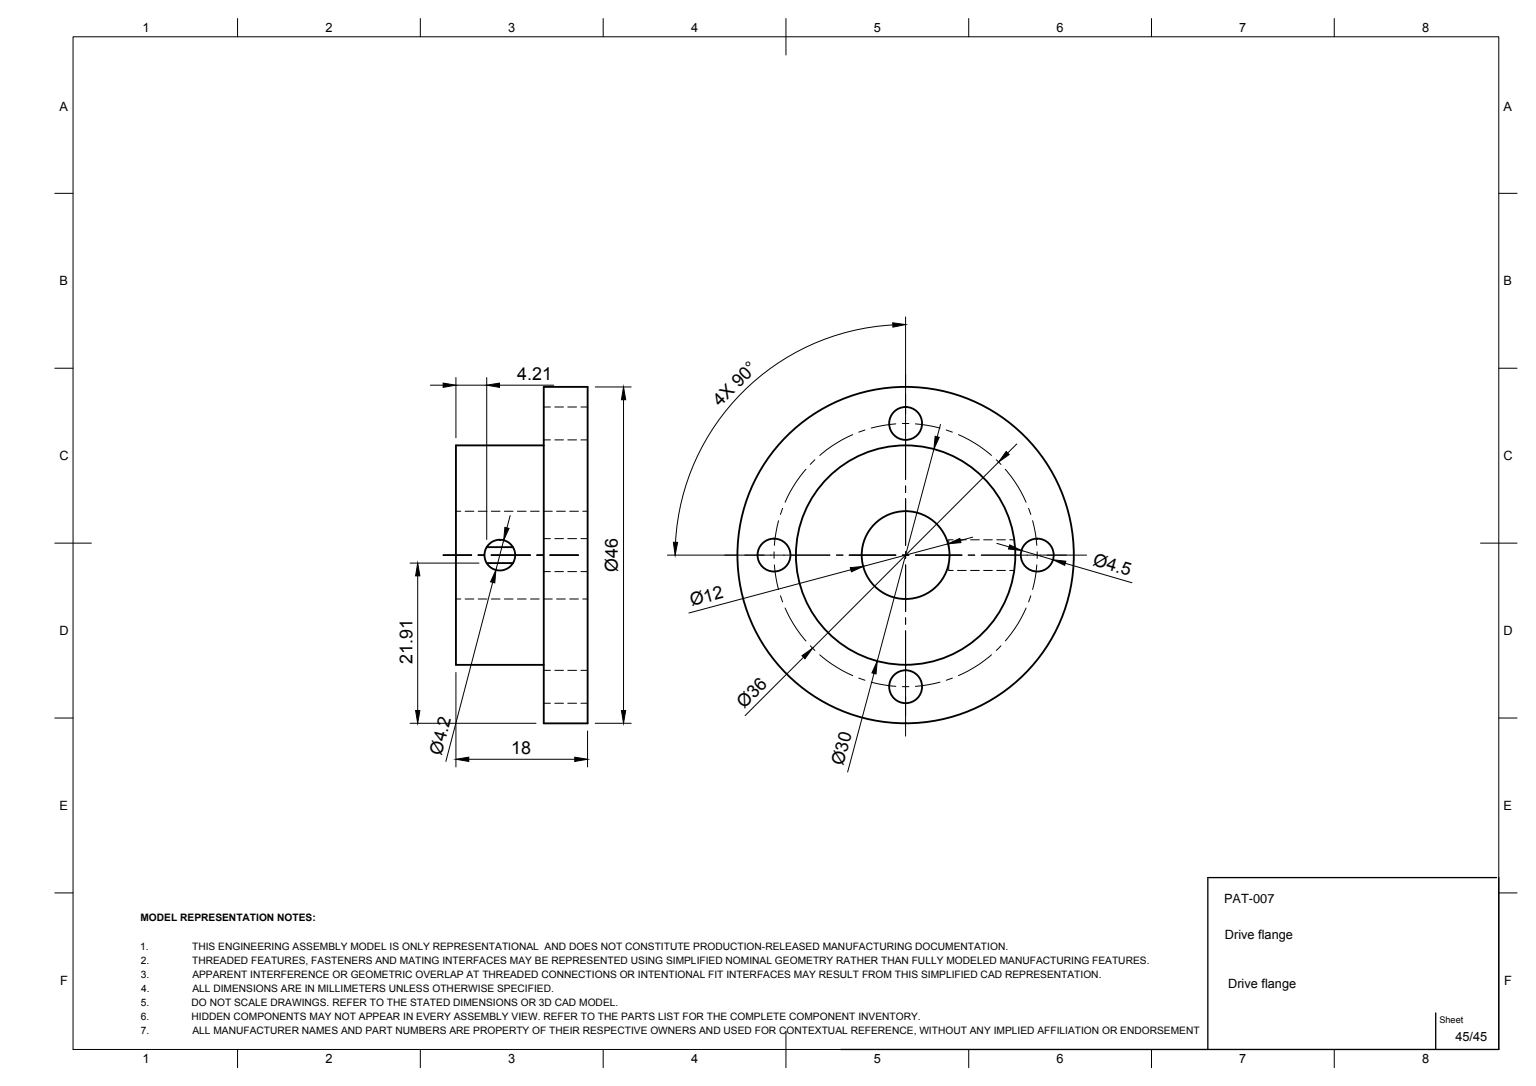
ISO-10303-21;
HEADER;
/* Generated by software containing ST-Developer
 * from STEP Tools, Inc. (www.steptools.com) 
 */

FILE_DESCRIPTION(
/* description */ ('Bearing friction torque test rig'),
/* implementation_level */ '2;1');

FILE_NAME(
/* name */ 'Drive flange.step',
/* time_stamp */ '2026-10-28T03:24:04-07:00',
/* author */ (''),
/* organization */ (''),
/* preprocessor_version */ 'ST-DEVELOPER v20.2',
/* originating_system */ 'Autodesk Translation Framework v15.17.0.0',
/* authorisation */ '');

FILE_SCHEMA (('AUTOMOTIVE_DESIGN { 1 0 10303 214 3 1 1 }'));
ENDSEC;

DATA;
#10=MECHANICAL_DESIGN_GEOMETRIC_PRESENTATION_REPRESENTATION('',(#591),#14822);
#391=B_SPLINE_CURVE_WITH_KNOTS('',3,(#14552,#14553,#14554,#14555,#14556,
#14557,#14558,#14559,#14560,#14561),.UNSPECIFIED.,.F.,.F.,(4,2,2,2,4),(0.847831445683407,
0.87827457693095,0.958092875386316,1.03791117384168,1.06835430508922),
 .UNSPECIFIED.);
#392=B_SPLINE_CURVE_WITH_KNOTS('',3,(#14567,#14568,#14569,#14570,#14571,
#14572,#14573,#14574,#14575,#14576,#14577,#14578,#14579,#14580,#14581,#14582,
#14583,#14584),.UNSPECIFIED.,.F.,.F.,(4,2,2,2,2,2,2,2,4),(0.,0.0792165807733633,
0.158433161546727,0.237648697074571,0.316864232602415,0.396079768130259,
0.475295303658104,0.554511884431467,0.63372846520483),.UNSPECIFIED.);
#393=B_SPLINE_CURVE_WITH_KNOTS('',3,(#14585,#14586,#14587,#14588,#14589,
#14590,#14591,#14592,#14593,#14594,#14595,#14596,#14597,#14598,#14599,#14600,
#14601,#14602),.UNSPECIFIED.,.F.,.F.,(4,2,2,2,2,2,2,2,4),(0.63372846520483,
0.712945045978194,0.792161626751557,0.871377162279401,0.950592697807245,
1.02980823333509,1.10902376886293,1.1882403496363,1.26745693040966),
 .UNSPECIFIED.);
#394=B_SPLINE_CURVE_WITH_KNOTS('',3,(#14605,#14606,#14607,#14608,#14609,
#14610,#14611,#14612,#14613,#14614),.UNSPECIFIED.,.F.,.F.,(4,2,2,2,4),(0.20910286209253,
0.239545993340073,0.319364291795439,0.399182590250804,0.429625721498348),
 .UNSPECIFIED.);
#498=SHAPE_REPRESENTATION_RELATIONSHIP('SRR','None',#15040,#537);
#537=ADVANCED_BREP_SHAPE_REPRESENTATION('',(#642),#14820);
#591=STYLED_ITEM('',(#15277),#642);
#642=MANIFOLD_SOLID_BREP('Body1',#7710);
#860=FACE_BOUND('',#2188,.T.);
#861=FACE_BOUND('',#2189,.T.);
#862=FACE_BOUND('',#2190,.T.);
#863=FACE_BOUND('',#2191,.T.);
#864=FACE_BOUND('',#2192,.T.);
#865=FACE_BOUND('',#2195,.T.);
#866=FACE_BOUND('',#2197,.T.);
#867=FACE_BOUND('',#2199,.T.);
#868=FACE_BOUND('',#2201,.T.);
#869=FACE_BOUND('',#2202,.T.);
#870=FACE_BOUND('',#2203,.T.);
#871=FACE_BOUND('',#2204,.T.);
#872=FACE_BOUND('',#2205,.T.);
#1085=PLANE('',#9102);
#1086=PLANE('',#9107);
#1087=PLANE('',#9120);
#1088=PLANE('',#9130);
#1089=PLANE('',#9131);
#1519=FACE_OUTER_BOUND('',#2180,.T.);
#1520=FACE_OUTER_BOUND('',#2181,.T.);
#1521=FACE_OUTER_BOUND('',#2182,.T.);
#1522=FACE_OUTER_BOUND('',#2183,.T.);
#1523=FACE_OUTER_BOUND('',#2184,.T.);
#1524=FACE_OUTER_BOUND('',#2185,.T.);
#1525=FACE_OUTER_BOUND('',#2186,.T.);
#1526=FACE_OUTER_BOUND('',#2187,.T.);
#1527=FACE_OUTER_BOUND('',#2193,.T.);
#1528=FACE_OUTER_BOUND('',#2194,.T.);
#1529=FACE_OUTER_BOUND('',#2196,.T.);
#1530=FACE_OUTER_BOUND('',#2198,.T.);
#1531=FACE_OUTER_BOUND('',#2200,.T.);
#2180=EDGE_LOOP('',(#6932,#6933));
#2181=EDGE_LOOP('',(#6934,#6935,#6936,#6937,#6938,#6939,#6940,#6941,#6942));
#2182=EDGE_LOOP('',(#6943,#6944,#6945));
#2183=EDGE_LOOP('',(#6946,#6947,#6948,#6949));
#2184=EDGE_LOOP('',(#6950,#6951,#6952,#6953));
#2185=EDGE_LOOP('',(#6954,#6955,#6956,#6957));
#2186=EDGE_LOOP('',(#6958,#6959,#6960,#6961));
#2187=EDGE_LOOP('',(#6962));
#2188=EDGE_LOOP('',(#6963));
#2189=EDGE_LOOP('',(#6964));
#2190=EDGE_LOOP('',(#6965));
#2191=EDGE_LOOP('',(#6966));
#2192=EDGE_LOOP('',(#6967));
#2193=EDGE_LOOP('',(#6968,#6969,#6970,#6971));
#2194=EDGE_LOOP('',(#6972,#6973,#6974,#6975));
#2195=EDGE_LOOP('',(#6976,#6977,#6978,#6979));
#2196=EDGE_LOOP('',(#6980,#6981,#6982,#6983));
#2197=EDGE_LOOP('',(#6984,#6985));
#2198=EDGE_LOOP('',(#6986));
#2199=EDGE_LOOP('',(#6987));
#2200=EDGE_LOOP('',(#6988));
#2201=EDGE_LOOP('',(#6989));
#2202=EDGE_LOOP('',(#6990));
#2203=EDGE_LOOP('',(#6991));
#2204=EDGE_LOOP('',(#6992));
#2205=EDGE_LOOP('',(#6993));
#2632=LINE('',#14548,#3076);
#2633=LINE('',#14565,#3077);
#2634=LINE('',#14616,#3078);
#2635=LINE('',#14621,#3079);
#2636=LINE('',#14627,#3080);
#2637=LINE('',#14633,#3081);
#2638=LINE('',#14639,#3082);
#2639=LINE('',#14648,#3083);
#2640=LINE('',#14654,#3084);
#2641=LINE('',#14659,#3085);
#3076=VECTOR('',#11501,1.);
#3077=VECTOR('',#11508,0.21);
#3078=VECTOR('',#11513,1.);
#3079=VECTOR('',#11518,0.225);
#3080=VECTOR('',#11525,0.225);
#3081=VECTOR('',#11532,0.225);
#3082=VECTOR('',#11539,0.225);
#3083=VECTOR('',#11550,2.3);
#3084=VECTOR('',#11557,0.6);
#3085=VECTOR('',#11564,1.5);
#3532=CIRCLE('',#9103,0.21);
#3533=CIRCLE('',#9105,0.21);
#3534=CIRCLE('',#9106,0.21);
#3535=CIRCLE('',#9109,0.225);
#3536=CIRCLE('',#9110,0.225);
#3537=CIRCLE('',#9112,0.225);
#3538=CIRCLE('',#9113,0.225);
#3539=CIRCLE('',#9115,0.225);
#3540=CIRCLE('',#9116,0.225);
#3541=CIRCLE('',#9118,0.225);
#3542=CIRCLE('',#9119,0.225);
#3543=CIRCLE('',#9121,2.3);
#3544=CIRCLE('',#9122,1.5);
#3545=CIRCLE('',#9124,2.3);
#3546=CIRCLE('',#9126,0.6);
#3547=CIRCLE('',#9127,0.6);
#3548=CIRCLE('',#9129,1.5);
#4163=VERTEX_POINT('',#14546);
#4164=VERTEX_POINT('',#14547);
#4165=VERTEX_POINT('',#14551);
#4166=VERTEX_POINT('',#14562);
#4167=VERTEX_POINT('',#14564);
#4168=VERTEX_POINT('',#14566);
#4169=VERTEX_POINT('',#14603);
#4170=VERTEX_POINT('',#14618);
#4171=VERTEX_POINT('',#14620);
#4172=VERTEX_POINT('',#14624);
#4173=VERTEX_POINT('',#14626);
#4174=VERTEX_POINT('',#14630);
#4175=VERTEX_POINT('',#14632);
#4176=VERTEX_POINT('',#14636);
#4177=VERTEX_POINT('',#14638);
#4178=VERTEX_POINT('',#14642);
#4179=VERTEX_POINT('',#14644);
#4180=VERTEX_POINT('',#14647);
#4181=VERTEX_POINT('',#14651);
#4182=VERTEX_POINT('',#14653);
#4183=VERTEX_POINT('',#14657);
#5092=EDGE_CURVE('',#4163,#4164,#2632,.T.);
#5093=EDGE_CURVE('',#4163,#4164,#3532,.T.);
#5094=EDGE_CURVE('',#4165,#4163,#391,.T.);
#5095=EDGE_CURVE('',#4166,#4165,#3533,.T.);
#5096=EDGE_CURVE('',#4166,#4167,#2633,.T.);
#5097=EDGE_CURVE('',#4168,#4167,#392,.T.);
#5098=EDGE_CURVE('',#4167,#4168,#393,.T.);
#5099=EDGE_CURVE('',#4169,#4166,#3534,.T.);
#5100=EDGE_CURVE('',#4164,#4169,#394,.T.);
#5101=EDGE_CURVE('',#4169,#4165,#2634,.T.);
#5102=EDGE_CURVE('',#4170,#4170,#3535,.T.);
#5103=EDGE_CURVE('',#4170,#4171,#2635,.T.);
#5104=EDGE_CURVE('',#4171,#4171,#3536,.T.);
#5105=EDGE_CURVE('',#4172,#4172,#3537,.T.);
#5106=EDGE_CURVE('',#4172,#4173,#2636,.T.);
#5107=EDGE_CURVE('',#4173,#4173,#3538,.T.);
#5108=EDGE_CURVE('',#4174,#4174,#3539,.T.);
#5109=EDGE_CURVE('',#4174,#4175,#2637,.T.);
#5110=EDGE_CURVE('',#4175,#4175,#3540,.T.);
#5111=EDGE_CURVE('',#4176,#4176,#3541,.T.);
#5112=EDGE_CURVE('',#4176,#4177,#2638,.T.);
#5113=EDGE_CURVE('',#4177,#4177,#3542,.T.);
#5114=EDGE_CURVE('',#4178,#4178,#3543,.T.);
#5115=EDGE_CURVE('',#4179,#4179,#3544,.T.);
#5116=EDGE_CURVE('',#4178,#4180,#2639,.T.);
#5117=EDGE_CURVE('',#4180,#4180,#3545,.T.);
#5118=EDGE_CURVE('',#4181,#4181,#3546,.T.);
#5119=EDGE_CURVE('',#4181,#4182,#2640,.T.);
#5120=EDGE_CURVE('',#4182,#4182,#3547,.T.);
#5121=EDGE_CURVE('',#4183,#4183,#3548,.T.);
#5122=EDGE_CURVE('',#4183,#4179,#2641,.T.);
#6932=ORIENTED_EDGE('',*,*,#5092,.F.);
#6933=ORIENTED_EDGE('',*,*,#5093,.T.);
#6934=ORIENTED_EDGE('',*,*,#5094,.F.);
#6935=ORIENTED_EDGE('',*,*,#5095,.F.);
#6936=ORIENTED_EDGE('',*,*,#5096,.T.);
#6937=ORIENTED_EDGE('',*,*,#5097,.F.);
#6938=ORIENTED_EDGE('',*,*,#5098,.F.);
#6939=ORIENTED_EDGE('',*,*,#5096,.F.);
#6940=ORIENTED_EDGE('',*,*,#5099,.F.);
#6941=ORIENTED_EDGE('',*,*,#5100,.F.);
#6942=ORIENTED_EDGE('',*,*,#5093,.F.);
#6943=ORIENTED_EDGE('',*,*,#5101,.F.);
#6944=ORIENTED_EDGE('',*,*,#5099,.T.);
#6945=ORIENTED_EDGE('',*,*,#5095,.T.);
#6946=ORIENTED_EDGE('',*,*,#5102,.F.);
#6947=ORIENTED_EDGE('',*,*,#5103,.T.);
#6948=ORIENTED_EDGE('',*,*,#5104,.F.);
#6949=ORIENTED_EDGE('',*,*,#5103,.F.);
#6950=ORIENTED_EDGE('',*,*,#5105,.F.);
#6951=ORIENTED_EDGE('',*,*,#5106,.T.);
#6952=ORIENTED_EDGE('',*,*,#5107,.F.);
#6953=ORIENTED_EDGE('',*,*,#5106,.F.);
#6954=ORIENTED_EDGE('',*,*,#5108,.F.);
#6955=ORIENTED_EDGE('',*,*,#5109,.T.);
#6956=ORIENTED_EDGE('',*,*,#5110,.F.);
#6957=ORIENTED_EDGE('',*,*,#5109,.F.);
#6958=ORIENTED_EDGE('',*,*,#5111,.F.);
#6959=ORIENTED_EDGE('',*,*,#5112,.T.);
#6960=ORIENTED_EDGE('',*,*,#5113,.F.);
#6961=ORIENTED_EDGE('',*,*,#5112,.F.);
#6962=ORIENTED_EDGE('',*,*,#5114,.T.);
#6963=ORIENTED_EDGE('',*,*,#5115,.F.);
#6964=ORIENTED_EDGE('',*,*,#5113,.T.);
#6965=ORIENTED_EDGE('',*,*,#5110,.T.);
#6966=ORIENTED_EDGE('',*,*,#5107,.T.);
#6967=ORIENTED_EDGE('',*,*,#5104,.T.);
#6968=ORIENTED_EDGE('',*,*,#5114,.F.);
#6969=ORIENTED_EDGE('',*,*,#5116,.T.);
#6970=ORIENTED_EDGE('',*,*,#5117,.T.);
#6971=ORIENTED_EDGE('',*,*,#5116,.F.);
#6972=ORIENTED_EDGE('',*,*,#5118,.F.);
#6973=ORIENTED_EDGE('',*,*,#5119,.T.);
#6974=ORIENTED_EDGE('',*,*,#5120,.T.);
#6975=ORIENTED_EDGE('',*,*,#5119,.F.);
#6976=ORIENTED_EDGE('',*,*,#5100,.T.);
#6977=ORIENTED_EDGE('',*,*,#5101,.T.);
#6978=ORIENTED_EDGE('',*,*,#5094,.T.);
#6979=ORIENTED_EDGE('',*,*,#5092,.T.);
#6980=ORIENTED_EDGE('',*,*,#5121,.F.);
#6981=ORIENTED_EDGE('',*,*,#5122,.T.);
#6982=ORIENTED_EDGE('',*,*,#5115,.T.);
#6983=ORIENTED_EDGE('',*,*,#5122,.F.);
#6984=ORIENTED_EDGE('',*,*,#5097,.T.);
#6985=ORIENTED_EDGE('',*,*,#5098,.T.);
#6986=ORIENTED_EDGE('',*,*,#5121,.T.);
#6987=ORIENTED_EDGE('',*,*,#5118,.T.);
#6988=ORIENTED_EDGE('',*,*,#5117,.F.);
#6989=ORIENTED_EDGE('',*,*,#5120,.F.);
#6990=ORIENTED_EDGE('',*,*,#5111,.T.);
#6991=ORIENTED_EDGE('',*,*,#5108,.T.);
#6992=ORIENTED_EDGE('',*,*,#5105,.T.);
#6993=ORIENTED_EDGE('',*,*,#5102,.T.);
#7201=CYLINDRICAL_SURFACE('',#9104,0.21);
#7202=CYLINDRICAL_SURFACE('',#9108,0.225);
#7203=CYLINDRICAL_SURFACE('',#9111,0.225);
#7204=CYLINDRICAL_SURFACE('',#9114,0.225);
#7205=CYLINDRICAL_SURFACE('',#9117,0.225);
#7206=CYLINDRICAL_SURFACE('',#9123,2.3);
#7207=CYLINDRICAL_SURFACE('',#9125,0.6);
#7208=CYLINDRICAL_SURFACE('',#9128,1.5);
#7630=ADVANCED_FACE('',(#1519),#1085,.T.);
#7631=ADVANCED_FACE('',(#1520),#7201,.F.);
#7632=ADVANCED_FACE('',(#1521),#1086,.T.);
#7633=ADVANCED_FACE('',(#1522),#7202,.F.);
#7634=ADVANCED_FACE('',(#1523),#7203,.F.);
#7635=ADVANCED_FACE('',(#1524),#7204,.F.);
#7636=ADVANCED_FACE('',(#1525),#7205,.F.);
#7637=ADVANCED_FACE('',(#1526,#860,#861,#862,#863,#864),#1087,.T.);
#7638=ADVANCED_FACE('',(#1527),#7206,.T.);
#7639=ADVANCED_FACE('',(#1528,#865),#7207,.F.);
#7640=ADVANCED_FACE('',(#1529,#866),#7208,.T.);
#7641=ADVANCED_FACE('',(#1530,#867),#1088,.T.);
#7642=ADVANCED_FACE('',(#1531,#868,#869,#870,#871,#872),#1089,.F.);
#7710=CLOSED_SHELL('',(#7630,#7631,#7632,#7633,#7634,#7635,#7636,#7637,
#7638,#7639,#7640,#7641,#7642));
#9101=AXIS2_PLACEMENT_3D('',#14544,#11497,#11498);
#9102=AXIS2_PLACEMENT_3D('',#14545,#11499,#11500);
#9103=AXIS2_PLACEMENT_3D('',#14549,#11502,#11503);
#9104=AXIS2_PLACEMENT_3D('',#14550,#11504,#11505);
#9105=AXIS2_PLACEMENT_3D('',#14563,#11506,#11507);
#9106=AXIS2_PLACEMENT_3D('',#14604,#11509,#11510);
#9107=AXIS2_PLACEMENT_3D('',#14615,#11511,#11512);
#9108=AXIS2_PLACEMENT_3D('',#14617,#11514,#11515);
#9109=AXIS2_PLACEMENT_3D('',#14619,#11516,#11517);
#9110=AXIS2_PLACEMENT_3D('',#14622,#11519,#11520);
#9111=AXIS2_PLACEMENT_3D('',#14623,#11521,#11522);
#9112=AXIS2_PLACEMENT_3D('',#14625,#11523,#11524);
#9113=AXIS2_PLACEMENT_3D('',#14628,#11526,#11527);
#9114=AXIS2_PLACEMENT_3D('',#14629,#11528,#11529);
#9115=AXIS2_PLACEMENT_3D('',#14631,#11530,#11531);
#9116=AXIS2_PLACEMENT_3D('',#14634,#11533,#11534);
#9117=AXIS2_PLACEMENT_3D('',#14635,#11535,#11536);
#9118=AXIS2_PLACEMENT_3D('',#14637,#11537,#11538);
#9119=AXIS2_PLACEMENT_3D('',#14640,#11540,#11541);
#9120=AXIS2_PLACEMENT_3D('',#14641,#11542,#11543);
#9121=AXIS2_PLACEMENT_3D('',#14643,#11544,#11545);
#9122=AXIS2_PLACEMENT_3D('',#14645,#11546,#11547);
#9123=AXIS2_PLACEMENT_3D('',#14646,#11548,#11549);
#9124=AXIS2_PLACEMENT_3D('',#14649,#11551,#11552);
#9125=AXIS2_PLACEMENT_3D('',#14650,#11553,#11554);
#9126=AXIS2_PLACEMENT_3D('',#14652,#11555,#11556);
#9127=AXIS2_PLACEMENT_3D('',#14655,#11558,#11559);
#9128=AXIS2_PLACEMENT_3D('',#14656,#11560,#11561);
#9129=AXIS2_PLACEMENT_3D('',#14658,#11562,#11563);
#9130=AXIS2_PLACEMENT_3D('',#14660,#11565,#11566);
#9131=AXIS2_PLACEMENT_3D('',#14661,#11567,#11568);
#11497=DIRECTION('axis',(0.,0.,1.));
#11498=DIRECTION('refdir',(1.,0.,0.));
#11499=DIRECTION('center_axis',(0.,0.,1.));
#11500=DIRECTION('ref_axis',(1.,0.,0.));
#11501=DIRECTION('',(0.,1.,0.));
#11502=DIRECTION('center_axis',(0.,0.,1.));
#11503=DIRECTION('ref_axis',(1.,0.,0.));
#11504=DIRECTION('center_axis',(0.,0.,1.));
#11505=DIRECTION('ref_axis',(1.,0.,0.));
#11506=DIRECTION('center_axis',(0.,0.,1.));
#11507=DIRECTION('ref_axis',(1.,0.,0.));
#11508=DIRECTION('',(0.,0.,1.));
#11509=DIRECTION('center_axis',(0.,0.,1.));
#11510=DIRECTION('ref_axis',(1.,0.,0.));
#11511=DIRECTION('center_axis',(0.,0.,1.));
#11512=DIRECTION('ref_axis',(1.,0.,0.));
#11513=DIRECTION('',(0.,-1.,0.));
#11514=DIRECTION('center_axis',(0.,1.,0.));
#11515=DIRECTION('ref_axis',(1.,0.,0.));
#11516=DIRECTION('center_axis',(0.,1.,0.));
#11517=DIRECTION('ref_axis',(1.,0.,0.));
#11518=DIRECTION('',(0.,1.,0.));
#11519=DIRECTION('center_axis',(0.,-1.,0.));
#11520=DIRECTION('ref_axis',(1.,0.,0.));
#11521=DIRECTION('center_axis',(0.,1.,0.));
#11522=DIRECTION('ref_axis',(1.,0.,0.));
#11523=DIRECTION('center_axis',(0.,1.,0.));
#11524=DIRECTION('ref_axis',(1.,0.,0.));
#11525=DIRECTION('',(0.,1.,0.));
#11526=DIRECTION('center_axis',(0.,-1.,0.));
#11527=DIRECTION('ref_axis',(1.,0.,0.));
#11528=DIRECTION('center_axis',(0.,1.,0.));
#11529=DIRECTION('ref_axis',(1.,0.,0.));
#11530=DIRECTION('center_axis',(0.,1.,0.));
#11531=DIRECTION('ref_axis',(1.,0.,0.));
#11532=DIRECTION('',(0.,1.,0.));
#11533=DIRECTION('center_axis',(0.,-1.,0.));
#11534=DIRECTION('ref_axis',(1.,0.,0.));
#11535=DIRECTION('center_axis',(0.,1.,0.));
#11536=DIRECTION('ref_axis',(1.,0.,0.));
#11537=DIRECTION('center_axis',(0.,1.,0.));
#11538=DIRECTION('ref_axis',(1.,0.,0.));
#11539=DIRECTION('',(0.,1.,0.));
#11540=DIRECTION('center_axis',(0.,-1.,0.));
#11541=DIRECTION('ref_axis',(1.,0.,0.));
#11542=DIRECTION('center_axis',(0.,1.,0.));
#11543=DIRECTION('ref_axis',(1.,0.,0.));
#11544=DIRECTION('center_axis',(0.,1.,0.));
#11545=DIRECTION('ref_axis',(1.,0.,0.));
#11546=DIRECTION('center_axis',(0.,1.,0.));
#11547=DIRECTION('ref_axis',(1.,0.,0.));
#11548=DIRECTION('center_axis',(0.,1.,0.));
#11549=DIRECTION('ref_axis',(1.,0.,0.));
#11550=DIRECTION('',(0.,-1.,0.));
#11551=DIRECTION('center_axis',(0.,1.,0.));
#11552=DIRECTION('ref_axis',(1.,0.,0.));
#11553=DIRECTION('center_axis',(0.,1.,0.));
#11554=DIRECTION('ref_axis',(1.,0.,0.));
#11555=DIRECTION('center_axis',(0.,-1.,0.));
#11556=DIRECTION('ref_axis',(1.,0.,0.));
#11557=DIRECTION('',(0.,-1.,0.));
#11558=DIRECTION('center_axis',(0.,-1.,0.));
#11559=DIRECTION('ref_axis',(1.,0.,0.));
#11560=DIRECTION('center_axis',(0.,1.,0.));
#11561=DIRECTION('ref_axis',(1.,0.,0.));
#11562=DIRECTION('center_axis',(0.,1.,0.));
#11563=DIRECTION('ref_axis',(1.,0.,0.));
#11564=DIRECTION('',(0.,-1.,0.));
#11565=DIRECTION('center_axis',(0.,1.,0.));
#11566=DIRECTION('ref_axis',(1.,0.,0.));
#11567=DIRECTION('center_axis',(0.,1.,0.));
#11568=DIRECTION('ref_axis',(1.,0.,0.));
#14544=CARTESIAN_POINT('',(0.,0.,0.));
#14545=CARTESIAN_POINT('Origin',(0.,-9.8,7.59));
#14546=CARTESIAN_POINT('',(0.109087121146353,-9.97944358444927,7.59));
#14547=CARTESIAN_POINT('',(0.109087121146353,-9.62055641555073,7.59));
#14548=CARTESIAN_POINT('',(0.109087121146353,-11.,7.59));
#14549=CARTESIAN_POINT('Origin',(0.,-9.8,7.59));
#14550=CARTESIAN_POINT('Origin',(0.,-9.8,7.59));
#14551=CARTESIAN_POINT('',(-0.109087121146353,-9.97944358444927,7.59));
#14552=CARTESIAN_POINT('Ctrl Pts',(-0.109087121146354,-9.97944358444927,
7.59));
#14553=CARTESIAN_POINT('Ctrl Pts',(-0.100058962329431,-9.98493197155217,
7.59166924721117));
#14554=CARTESIAN_POINT('Ctrl Pts',(-0.0905297208284648,-9.98978489888129,
7.59321436338553));
#14555=CARTESIAN_POINT('Ctrl Pts',(-0.0548356965671429,-10.0046369707595,
7.598057680137));
#14556=CARTESIAN_POINT('Ctrl Pts',(-0.026606099485122,-10.01,7.6));
#14557=CARTESIAN_POINT('Ctrl Pts',(0.0266060994851219,-10.01,7.6));
#14558=CARTESIAN_POINT('Ctrl Pts',(0.0548356965671429,-10.0046369707595,
7.598057680137));
#14559=CARTESIAN_POINT('Ctrl Pts',(0.0905297208284645,-9.98978489888129,
7.59321436338553));
#14560=CARTESIAN_POINT('Ctrl Pts',(0.100058962329432,-9.98493197155217,
7.59166924721117));
#14561=CARTESIAN_POINT('Ctrl Pts',(0.109087121146353,-9.97944358444927,
7.59));
#14562=CARTESIAN_POINT('',(-0.21,-9.8,7.59));
#14563=CARTESIAN_POINT('Origin',(0.,-9.8,7.59));
#14564=CARTESIAN_POINT('',(-0.21,-9.8,8.48522725533839));
#14565=CARTESIAN_POINT('',(-0.21,-9.8,7.59));
#14566=CARTESIAN_POINT('',(0.21,-9.8,8.48522725533839));
#14567=CARTESIAN_POINT('Ctrl Pts',(0.21,-9.8,8.48522725533839));
#14568=CARTESIAN_POINT('Ctrl Pts',(0.21,-9.82640552692446,8.48522725533839));
#14569=CARTESIAN_POINT('Ctrl Pts',(0.204715737269595,-9.85454707409072,
8.48600415954412));
#14570=CARTESIAN_POINT('Ctrl Pts',(0.183273763036331,-9.90627626890513,
8.48880073282317));
#14571=CARTESIAN_POINT('Ctrl Pts',(0.167117923970394,-9.92986692412796,
8.49077897157582));
#14572=CARTESIAN_POINT('Ctrl Pts',(0.129867169887369,-9.96711767821098,
8.49448481141327));
#14573=CARTESIAN_POINT('Ctrl Pts',(0.106276408305765,-9.98327371000135,
8.49645455657129));
#14574=CARTESIAN_POINT('Ctrl Pts',(0.0545468514059001,-10.0047158248262,
8.49923165515646));
#14575=CARTESIAN_POINT('Ctrl Pts',(0.0264051785092814,-10.01,8.5));
#14576=CARTESIAN_POINT('Ctrl Pts',(-0.0264051785092814,-10.01,8.5));
#14577=CARTESIAN_POINT('Ctrl Pts',(-0.0545468514058994,-10.0047158248262,
8.49923165515646));
#14578=CARTESIAN_POINT('Ctrl Pts',(-0.106276408305765,-9.98327371000135,
8.49645455657129));
#14579=CARTESIAN_POINT('Ctrl Pts',(-0.129867169887368,-9.96711767821098,
8.49448481141327));
#14580=CARTESIAN_POINT('Ctrl Pts',(-0.167117923970393,-9.92986692412796,
8.49077897157582));
#14581=CARTESIAN_POINT('Ctrl Pts',(-0.183273763036331,-9.90627626890513,
8.48880073282317));
#14582=CARTESIAN_POINT('Ctrl Pts',(-0.204715737269595,-9.85454707409072,
8.48600415954412));
#14583=CARTESIAN_POINT('Ctrl Pts',(-0.21,-9.82640552692446,8.48522725533839));
#14584=CARTESIAN_POINT('Ctrl Pts',(-0.21,-9.8,8.48522725533839));
#14585=CARTESIAN_POINT('Ctrl Pts',(-0.21,-9.8,8.48522725533839));
#14586=CARTESIAN_POINT('Ctrl Pts',(-0.21,-9.77359447307554,8.48522725533839));
#14587=CARTESIAN_POINT('Ctrl Pts',(-0.204715737269595,-9.74545292590929,
8.48600415954412));
#14588=CARTESIAN_POINT('Ctrl Pts',(-0.183273763036331,-9.69372373109487,
8.48880073282317));
#14589=CARTESIAN_POINT('Ctrl Pts',(-0.167117923970394,-9.67013307587204,
8.49077897157582));
#14590=CARTESIAN_POINT('Ctrl Pts',(-0.129867169887369,-9.63288232178902,
8.49448481141327));
#14591=CARTESIAN_POINT('Ctrl Pts',(-0.106276408305765,-9.61672628999865,
8.49645455657129));
#14592=CARTESIAN_POINT('Ctrl Pts',(-0.0545468514059001,-9.59528417517378,
8.49923165515646));
#14593=CARTESIAN_POINT('Ctrl Pts',(-0.0264051785092815,-9.59,8.5));
#14594=CARTESIAN_POINT('Ctrl Pts',(0.0264051785092813,-9.59,8.5));
#14595=CARTESIAN_POINT('Ctrl Pts',(0.0545468514058994,-9.59528417517378,
8.49923165515645));
#14596=CARTESIAN_POINT('Ctrl Pts',(0.106276408305765,-9.61672628999865,
8.49645455657129));
#14597=CARTESIAN_POINT('Ctrl Pts',(0.129867169887368,-9.63288232178902,
8.49448481141327));
#14598=CARTESIAN_POINT('Ctrl Pts',(0.167117923970393,-9.67013307587204,
8.49077897157582));
#14599=CARTESIAN_POINT('Ctrl Pts',(0.183273763036331,-9.69372373109487,
8.48880073282317));
#14600=CARTESIAN_POINT('Ctrl Pts',(0.204715737269595,-9.74545292590929,
8.48600415954412));
#14601=CARTESIAN_POINT('Ctrl Pts',(0.21,-9.77359447307554,8.48522725533839));
#14602=CARTESIAN_POINT('Ctrl Pts',(0.21,-9.8,8.48522725533839));
#14603=CARTESIAN_POINT('',(-0.109087121146353,-9.62055641555073,7.59));
#14604=CARTESIAN_POINT('Origin',(0.,-9.8,7.59));
#14605=CARTESIAN_POINT('Ctrl Pts',(0.109087121146353,-9.62055641555074,
7.59));
#14606=CARTESIAN_POINT('Ctrl Pts',(0.100058962329431,-9.61506802844783,
7.59166924721117));
#14607=CARTESIAN_POINT('Ctrl Pts',(0.0905297208284649,-9.61021510111872,
7.59321436338553));
#14608=CARTESIAN_POINT('Ctrl Pts',(0.054835696567143,-9.59536302924048,
7.598057680137));
#14609=CARTESIAN_POINT('Ctrl Pts',(0.026606099485122,-9.59,7.6));
#14610=CARTESIAN_POINT('Ctrl Pts',(-0.026606099485122,-9.59,7.6));
#14611=CARTESIAN_POINT('Ctrl Pts',(-0.0548356965671429,-9.59536302924048,
7.598057680137));
#14612=CARTESIAN_POINT('Ctrl Pts',(-0.090529720828465,-9.61021510111872,
7.59321436338553));
#14613=CARTESIAN_POINT('Ctrl Pts',(-0.100058962329431,-9.61506802844783,
7.59166924721117));
#14614=CARTESIAN_POINT('Ctrl Pts',(-0.109087121146353,-9.62055641555073,
7.59));
#14615=CARTESIAN_POINT('Origin',(0.,-9.8,7.59));
#14616=CARTESIAN_POINT('',(-0.109087121146353,-11.,7.59));
#14617=CARTESIAN_POINT('Origin',(-1.8,-11.1,7.));
#14618=CARTESIAN_POINT('',(-2.025,-11.,7.));
#14619=CARTESIAN_POINT('Origin',(-1.8,-11.,7.));
#14620=CARTESIAN_POINT('',(-2.025,-10.4,7.));
#14621=CARTESIAN_POINT('',(-2.025,-11.1,7.));
#14622=CARTESIAN_POINT('Origin',(-1.8,-10.4,7.));
#14623=CARTESIAN_POINT('Origin',(1.10218211923262E-16,-11.1,8.8));
#14624=CARTESIAN_POINT('',(-0.225,-11.,8.8));
#14625=CARTESIAN_POINT('Origin',(1.10218211923262E-16,-11.,8.8));
#14626=CARTESIAN_POINT('',(-0.225,-10.4,8.8));
#14627=CARTESIAN_POINT('',(-0.225,-11.1,8.8));
#14628=CARTESIAN_POINT('Origin',(1.10218211923262E-16,-10.4,8.8));
#14629=CARTESIAN_POINT('Origin',(1.8,-11.1,7.));
#14630=CARTESIAN_POINT('',(1.575,-11.,7.));
#14631=CARTESIAN_POINT('Origin',(1.8,-11.,7.));
#14632=CARTESIAN_POINT('',(1.575,-10.4,7.));
#14633=CARTESIAN_POINT('',(1.575,-11.1,7.));
#14634=CARTESIAN_POINT('Origin',(1.8,-10.4,7.));
#14635=CARTESIAN_POINT('Origin',(-3.30654635769785E-16,-11.1,5.2));
#14636=CARTESIAN_POINT('',(-0.225,-11.,5.2));
#14637=CARTESIAN_POINT('Origin',(-3.30654635769785E-16,-11.,5.2));
#14638=CARTESIAN_POINT('',(-0.225,-10.4,5.2));
#14639=CARTESIAN_POINT('',(-0.225,-11.1,5.2));
#14640=CARTESIAN_POINT('Origin',(-3.30654635769785E-16,-10.4,5.2));
#14641=CARTESIAN_POINT('Origin',(0.,-10.4,7.));
#14642=CARTESIAN_POINT('',(-2.3,-10.4,7.));
#14643=CARTESIAN_POINT('Origin',(0.,-10.4,7.));
#14644=CARTESIAN_POINT('',(-1.5,-10.4,7.));
#14645=CARTESIAN_POINT('Origin',(0.,-10.4,7.));
#14646=CARTESIAN_POINT('Origin',(0.,-11.,7.));
#14647=CARTESIAN_POINT('',(-2.3,-11.,7.));
#14648=CARTESIAN_POINT('',(-2.3,-11.,7.));
#14649=CARTESIAN_POINT('Origin',(0.,-11.,7.));
#14650=CARTESIAN_POINT('Origin',(0.,-11.,7.));
#14651=CARTESIAN_POINT('',(-0.6,-9.2,7.));
#14652=CARTESIAN_POINT('Origin',(0.,-9.2,7.));
#14653=CARTESIAN_POINT('',(-0.6,-11.,7.));
#14654=CARTESIAN_POINT('',(-0.6,-11.,7.));
#14655=CARTESIAN_POINT('Origin',(0.,-11.,7.));
#14656=CARTESIAN_POINT('Origin',(0.,-11.,7.));
#14657=CARTESIAN_POINT('',(-1.5,-9.2,7.));
#14658=CARTESIAN_POINT('Origin',(0.,-9.2,7.));
#14659=CARTESIAN_POINT('',(-1.5,-11.,7.));
#14660=CARTESIAN_POINT('Origin',(0.,-9.2,7.));
#14661=CARTESIAN_POINT('Origin',(0.,-11.,7.));
#14775=UNCERTAINTY_MEASURE_WITH_UNIT(LENGTH_MEASURE(0.001),#14823,
'DISTANCE_ACCURACY_VALUE',
'Maximum model space distance between geometric entities at asserted c
onnectivities');
#14777=UNCERTAINTY_MEASURE_WITH_UNIT(LENGTH_MEASURE(0.001),#14823,
'DISTANCE_ACCURACY_VALUE',
'Maximum model space distance between geometric entities at asserted c
onnectivities');
#14820=(
GEOMETRIC_REPRESENTATION_CONTEXT(3)
GLOBAL_UNCERTAINTY_ASSIGNED_CONTEXT((#14775))
GLOBAL_UNIT_ASSIGNED_CONTEXT((#14823,#14825,#14826))
REPRESENTATION_CONTEXT('','3D')
);
#14822=(
GEOMETRIC_REPRESENTATION_CONTEXT(3)
GLOBAL_UNCERTAINTY_ASSIGNED_CONTEXT((#14777))
GLOBAL_UNIT_ASSIGNED_CONTEXT((#14823,#14825,#14826))
REPRESENTATION_CONTEXT('','3D')
);
#14823=(
LENGTH_UNIT()
NAMED_UNIT(*)
SI_UNIT(.CENTI.,.METRE.)
);
#14825=(
NAMED_UNIT(*)
PLANE_ANGLE_UNIT()
SI_UNIT($,.RADIAN.)
);
#14826=(
NAMED_UNIT(*)
SI_UNIT($,.STERADIAN.)
SOLID_ANGLE_UNIT()
);
#14869=SHAPE_DEFINITION_REPRESENTATION(#14979,#15040);
#14979=PRODUCT_DEFINITION_SHAPE('',$,#15085);
#15040=SHAPE_REPRESENTATION('',(#9101),#14820);
#15042=PRODUCT_DEFINITION_CONTEXT('part definition',#15176,'design');
#15085=PRODUCT_DEFINITION('Drive flange','Drive flange',#15129,#15042);
#15129=PRODUCT_DEFINITION_FORMATION('',$,#15220);
#15176=APPLICATION_CONTEXT(
'Core Data for Automotive Mechanical Design Process');
#15177=PRODUCT_CONTEXT('part definition',#15176,'mechanical');
#15220=PRODUCT('Drive flange','Drive flange','Drive flange',(#15177));
#15271=COLOUR_RGB('Sky Blue',0.24,0.69,0.87);
#15272=FILL_AREA_STYLE_COLOUR('',#15271);
#15273=FILL_AREA_STYLE('',(#15272));
#15274=SURFACE_STYLE_FILL_AREA(#15273);
#15275=SURFACE_SIDE_STYLE('',(#15274));
#15276=SURFACE_STYLE_USAGE(.BOTH.,#15275);
#15277=PRESENTATION_STYLE_ASSIGNMENT((#15276));
ENDSEC;
END-ISO-10303-21;
